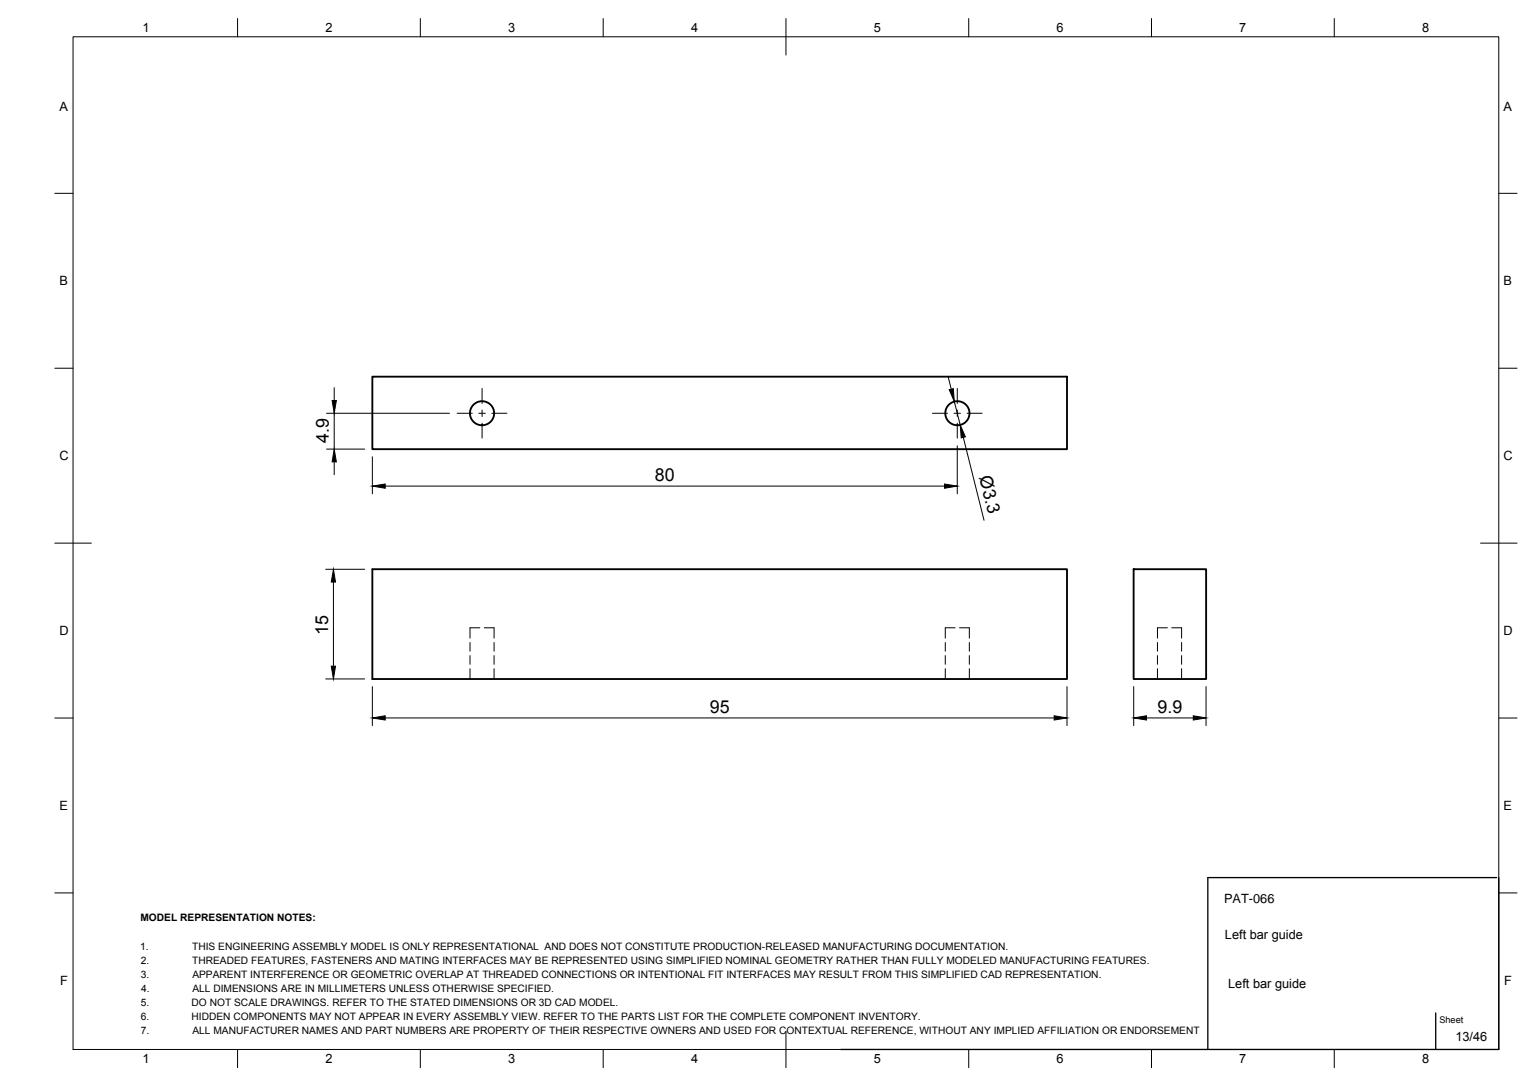
ISO-10303-21;
HEADER;
/* Generated by software containing ST-Developer
 * from STEP Tools, Inc. (www.steptools.com) 
 */

FILE_DESCRIPTION(
/* description */ ('Lever-operated bar clamp (toggle)'),
/* implementation_level */ '2;1');

FILE_NAME(
/* name */ 'Left bar guide.step',
/* time_stamp */ '2026-10-28T03:25:02-07:00',
/* author */ (''),
/* organization */ (''),
/* preprocessor_version */ 'ST-DEVELOPER v20.2',
/* originating_system */ 'Autodesk Translation Framework v15.17.0.0',
/* authorisation */ '');

FILE_SCHEMA (('AUTOMOTIVE_DESIGN { 1 0 10303 214 3 1 1 }'));
ENDSEC;

DATA;
#10=MECHANICAL_DESIGN_GEOMETRIC_PRESENTATION_REPRESENTATION('',(#418),#12413);
#342=SHAPE_REPRESENTATION_RELATIONSHIP('SRR','None',#12581,#380);
#380=ADVANCED_BREP_SHAPE_REPRESENTATION('',(#465),#12378);
#418=STYLED_ITEM('',(#12862),#465);
#465=MANIFOLD_SOLID_BREP('Body1',#6577);
#581=FACE_BOUND('',#1493,.T.);
#582=FACE_BOUND('',#1494,.T.);
#708=PLANE('',#7263);
#709=PLANE('',#7267);
#710=PLANE('',#7268);
#711=PLANE('',#7269);
#712=PLANE('',#7270);
#713=PLANE('',#7271);
#714=PLANE('',#7272);
#715=PLANE('',#7273);
#996=FACE_OUTER_BOUND('',#1483,.T.);
#997=FACE_OUTER_BOUND('',#1484,.T.);
#998=FACE_OUTER_BOUND('',#1485,.T.);
#999=FACE_OUTER_BOUND('',#1486,.T.);
#1000=FACE_OUTER_BOUND('',#1487,.T.);
#1001=FACE_OUTER_BOUND('',#1488,.T.);
#1002=FACE_OUTER_BOUND('',#1489,.T.);
#1003=FACE_OUTER_BOUND('',#1490,.T.);
#1004=FACE_OUTER_BOUND('',#1491,.T.);
#1005=FACE_OUTER_BOUND('',#1492,.T.);
#1483=EDGE_LOOP('',(#4895,#4896,#4897,#4898));
#1484=EDGE_LOOP('',(#4899));
#1485=EDGE_LOOP('',(#4900,#4901,#4902,#4903));
#1486=EDGE_LOOP('',(#4904));
#1487=EDGE_LOOP('',(#4905,#4906,#4907,#4908));
#1488=EDGE_LOOP('',(#4909,#4910,#4911,#4912));
#1489=EDGE_LOOP('',(#4913,#4914,#4915,#4916));
#1490=EDGE_LOOP('',(#4917,#4918,#4919,#4920));
#1491=EDGE_LOOP('',(#4921,#4922,#4923,#4924));
#1492=EDGE_LOOP('',(#4925,#4926,#4927,#4928));
#1493=EDGE_LOOP('',(#4929));
#1494=EDGE_LOOP('',(#4930));
#1986=LINE('',#10563,#2427);
#1987=LINE('',#10570,#2428);
#1988=LINE('',#10576,#2429);
#1989=LINE('',#10578,#2430);
#1990=LINE('',#10580,#2431);
#1991=LINE('',#10581,#2432);
#1992=LINE('',#10584,#2433);
#1993=LINE('',#10586,#2434);
#1994=LINE('',#10587,#2435);
#1995=LINE('',#10590,#2436);
#1996=LINE('',#10592,#2437);
#1997=LINE('',#10593,#2438);
#1998=LINE('',#10595,#2439);
#1999=LINE('',#10596,#2440);
#2427=VECTOR('',#8475,0.165);
#2428=VECTOR('',#8484,0.165);
#2429=VECTOR('',#8491,1.);
#2430=VECTOR('',#8492,1.);
#2431=VECTOR('',#8493,1.);
#2432=VECTOR('',#8494,1.);
#2433=VECTOR('',#8497,1.);
#2434=VECTOR('',#8498,1.);
#2435=VECTOR('',#8499,1.);
#2436=VECTOR('',#8502,1.);
#2437=VECTOR('',#8503,1.);
#2438=VECTOR('',#8504,1.);
#2439=VECTOR('',#8507,1.);
#2440=VECTOR('',#8508,1.);
#2835=CIRCLE('',#7261,0.165);
#2836=CIRCLE('',#7262,0.165);
#2837=CIRCLE('',#7265,0.165);
#2838=CIRCLE('',#7266,0.165);
#3232=VERTEX_POINT('',#10560);
#3233=VERTEX_POINT('',#10562);
#3234=VERTEX_POINT('',#10567);
#3235=VERTEX_POINT('',#10569);
#3236=VERTEX_POINT('',#10574);
#3237=VERTEX_POINT('',#10575);
#3238=VERTEX_POINT('',#10577);
#3239=VERTEX_POINT('',#10579);
#3240=VERTEX_POINT('',#10583);
#3241=VERTEX_POINT('',#10585);
#3242=VERTEX_POINT('',#10589);
#3243=VERTEX_POINT('',#10591);
#3852=EDGE_CURVE('',#3232,#3232,#2835,.T.);
#3853=EDGE_CURVE('',#3232,#3233,#1986,.T.);
#3854=EDGE_CURVE('',#3233,#3233,#2836,.T.);
#3855=EDGE_CURVE('',#3234,#3234,#2837,.T.);
#3856=EDGE_CURVE('',#3234,#3235,#1987,.T.);
#3857=EDGE_CURVE('',#3235,#3235,#2838,.T.);
#3858=EDGE_CURVE('',#3236,#3237,#1988,.T.);
#3859=EDGE_CURVE('',#3237,#3238,#1989,.T.);
#3860=EDGE_CURVE('',#3239,#3238,#1990,.T.);
#3861=EDGE_CURVE('',#3236,#3239,#1991,.T.);
#3862=EDGE_CURVE('',#3240,#3236,#1992,.T.);
#3863=EDGE_CURVE('',#3241,#3239,#1993,.T.);
#3864=EDGE_CURVE('',#3240,#3241,#1994,.T.);
#3865=EDGE_CURVE('',#3242,#3240,#1995,.T.);
#3866=EDGE_CURVE('',#3243,#3241,#1996,.T.);
#3867=EDGE_CURVE('',#3242,#3243,#1997,.T.);
#3868=EDGE_CURVE('',#3237,#3242,#1998,.T.);
#3869=EDGE_CURVE('',#3238,#3243,#1999,.T.);
#4895=ORIENTED_EDGE('',*,*,#3852,.F.);
#4896=ORIENTED_EDGE('',*,*,#3853,.T.);
#4897=ORIENTED_EDGE('',*,*,#3854,.T.);
#4898=ORIENTED_EDGE('',*,*,#3853,.F.);
#4899=ORIENTED_EDGE('',*,*,#3854,.F.);
#4900=ORIENTED_EDGE('',*,*,#3855,.F.);
#4901=ORIENTED_EDGE('',*,*,#3856,.T.);
#4902=ORIENTED_EDGE('',*,*,#3857,.T.);
#4903=ORIENTED_EDGE('',*,*,#3856,.F.);
#4904=ORIENTED_EDGE('',*,*,#3857,.F.);
#4905=ORIENTED_EDGE('',*,*,#3858,.T.);
#4906=ORIENTED_EDGE('',*,*,#3859,.T.);
#4907=ORIENTED_EDGE('',*,*,#3860,.F.);
#4908=ORIENTED_EDGE('',*,*,#3861,.F.);
#4909=ORIENTED_EDGE('',*,*,#3862,.T.);
#4910=ORIENTED_EDGE('',*,*,#3861,.T.);
#4911=ORIENTED_EDGE('',*,*,#3863,.F.);
#4912=ORIENTED_EDGE('',*,*,#3864,.F.);
#4913=ORIENTED_EDGE('',*,*,#3865,.T.);
#4914=ORIENTED_EDGE('',*,*,#3864,.T.);
#4915=ORIENTED_EDGE('',*,*,#3866,.F.);
#4916=ORIENTED_EDGE('',*,*,#3867,.F.);
#4917=ORIENTED_EDGE('',*,*,#3868,.T.);
#4918=ORIENTED_EDGE('',*,*,#3867,.T.);
#4919=ORIENTED_EDGE('',*,*,#3869,.F.);
#4920=ORIENTED_EDGE('',*,*,#3859,.F.);
#4921=ORIENTED_EDGE('',*,*,#3869,.T.);
#4922=ORIENTED_EDGE('',*,*,#3866,.T.);
#4923=ORIENTED_EDGE('',*,*,#3863,.T.);
#4924=ORIENTED_EDGE('',*,*,#3860,.T.);
#4925=ORIENTED_EDGE('',*,*,#3868,.F.);
#4926=ORIENTED_EDGE('',*,*,#3858,.F.);
#4927=ORIENTED_EDGE('',*,*,#3862,.F.);
#4928=ORIENTED_EDGE('',*,*,#3865,.F.);
#4929=ORIENTED_EDGE('',*,*,#3852,.T.);
#4930=ORIENTED_EDGE('',*,*,#3855,.T.);
#6084=CYLINDRICAL_SURFACE('',#7260,0.165);
#6085=CYLINDRICAL_SURFACE('',#7264,0.165);
#6271=ADVANCED_FACE('',(#996),#6084,.F.);
#6272=ADVANCED_FACE('',(#997),#708,.F.);
#6273=ADVANCED_FACE('',(#998),#6085,.F.);
#6274=ADVANCED_FACE('',(#999),#709,.F.);
#6275=ADVANCED_FACE('',(#1000),#710,.T.);
#6276=ADVANCED_FACE('',(#1001),#711,.T.);
#6277=ADVANCED_FACE('',(#1002),#712,.T.);
#6278=ADVANCED_FACE('',(#1003),#713,.T.);
#6279=ADVANCED_FACE('',(#1004),#714,.T.);
#6280=ADVANCED_FACE('',(#1005,#581,#582),#715,.F.);
#6577=CLOSED_SHELL('',(#6271,#6272,#6273,#6274,#6275,#6276,#6277,#6278,
#6279,#6280));
#7259=AXIS2_PLACEMENT_3D('',#10558,#8469,#8470);
#7260=AXIS2_PLACEMENT_3D('',#10559,#8471,#8472);
#7261=AXIS2_PLACEMENT_3D('',#10561,#8473,#8474);
#7262=AXIS2_PLACEMENT_3D('',#10564,#8476,#8477);
#7263=AXIS2_PLACEMENT_3D('',#10565,#8478,#8479);
#7264=AXIS2_PLACEMENT_3D('',#10566,#8480,#8481);
#7265=AXIS2_PLACEMENT_3D('',#10568,#8482,#8483);
#7266=AXIS2_PLACEMENT_3D('',#10571,#8485,#8486);
#7267=AXIS2_PLACEMENT_3D('',#10572,#8487,#8488);
#7268=AXIS2_PLACEMENT_3D('',#10573,#8489,#8490);
#7269=AXIS2_PLACEMENT_3D('',#10582,#8495,#8496);
#7270=AXIS2_PLACEMENT_3D('',#10588,#8500,#8501);
#7271=AXIS2_PLACEMENT_3D('',#10594,#8505,#8506);
#7272=AXIS2_PLACEMENT_3D('',#10597,#8509,#8510);
#7273=AXIS2_PLACEMENT_3D('',#10598,#8511,#8512);
#8469=DIRECTION('axis',(0.,0.,1.));
#8470=DIRECTION('refdir',(1.,0.,0.));
#8471=DIRECTION('center_axis',(0.,0.,1.));
#8472=DIRECTION('ref_axis',(1.,0.,0.));
#8473=DIRECTION('center_axis',(0.,0.,1.));
#8474=DIRECTION('ref_axis',(1.,0.,0.));
#8475=DIRECTION('',(0.,0.,1.));
#8476=DIRECTION('center_axis',(0.,0.,1.));
#8477=DIRECTION('ref_axis',(1.,0.,0.));
#8478=DIRECTION('center_axis',(0.,0.,1.));
#8479=DIRECTION('ref_axis',(1.,0.,0.));
#8480=DIRECTION('center_axis',(0.,0.,1.));
#8481=DIRECTION('ref_axis',(1.,0.,0.));
#8482=DIRECTION('center_axis',(0.,0.,1.));
#8483=DIRECTION('ref_axis',(1.,0.,0.));
#8484=DIRECTION('',(0.,0.,1.));
#8485=DIRECTION('center_axis',(0.,0.,1.));
#8486=DIRECTION('ref_axis',(1.,0.,0.));
#8487=DIRECTION('center_axis',(0.,0.,1.));
#8488=DIRECTION('ref_axis',(1.,0.,0.));
#8489=DIRECTION('center_axis',(0.,1.,0.));
#8490=DIRECTION('ref_axis',(-1.,0.,0.));
#8491=DIRECTION('',(-1.,0.,0.));
#8492=DIRECTION('',(0.,0.,1.));
#8493=DIRECTION('',(-1.,0.,0.));
#8494=DIRECTION('',(0.,0.,1.));
#8495=DIRECTION('center_axis',(1.,0.,0.));
#8496=DIRECTION('ref_axis',(0.,1.,0.));
#8497=DIRECTION('',(0.,1.,0.));
#8498=DIRECTION('',(0.,1.,0.));
#8499=DIRECTION('',(0.,0.,1.));
#8500=DIRECTION('center_axis',(0.,-1.,0.));
#8501=DIRECTION('ref_axis',(1.,0.,0.));
#8502=DIRECTION('',(1.,0.,0.));
#8503=DIRECTION('',(1.,0.,0.));
#8504=DIRECTION('',(0.,0.,1.));
#8505=DIRECTION('center_axis',(-1.,0.,0.));
#8506=DIRECTION('ref_axis',(0.,-1.,0.));
#8507=DIRECTION('',(0.,-1.,0.));
#8508=DIRECTION('',(0.,-1.,0.));
#8509=DIRECTION('center_axis',(0.,0.,1.));
#8510=DIRECTION('ref_axis',(1.,0.,0.));
#8511=DIRECTION('center_axis',(0.,0.,1.));
#8512=DIRECTION('ref_axis',(1.,0.,0.));
#10558=CARTESIAN_POINT('',(0.,0.,0.));
#10559=CARTESIAN_POINT('Origin',(-1.5,-4.5,0.9));
#10560=CARTESIAN_POINT('',(-1.665,-4.5,1.));
#10561=CARTESIAN_POINT('Origin',(-1.5,-4.5,1.));
#10562=CARTESIAN_POINT('',(-1.665,-4.5,1.7));
#10563=CARTESIAN_POINT('',(-1.665,-4.5,0.9));
#10564=CARTESIAN_POINT('Origin',(-1.5,-4.5,1.7));
#10565=CARTESIAN_POINT('Origin',(-1.5,-4.5,1.7));
#10566=CARTESIAN_POINT('Origin',(-1.5,2.,0.9));
#10567=CARTESIAN_POINT('',(-1.665,2.,1.));
#10568=CARTESIAN_POINT('Origin',(-1.5,2.,1.));
#10569=CARTESIAN_POINT('',(-1.665,2.,1.7));
#10570=CARTESIAN_POINT('',(-1.665,2.,0.9));
#10571=CARTESIAN_POINT('Origin',(-1.5,2.,1.7));
#10572=CARTESIAN_POINT('Origin',(-1.5,2.,1.7));
#10573=CARTESIAN_POINT('Origin',(-1.01,3.5,1.));
#10574=CARTESIAN_POINT('',(-1.01,3.5,1.));
#10575=CARTESIAN_POINT('',(-2.,3.5,1.));
#10576=CARTESIAN_POINT('',(-1.01,3.5,1.));
#10577=CARTESIAN_POINT('',(-2.,3.5,2.5));
#10578=CARTESIAN_POINT('',(-2.,3.5,1.));
#10579=CARTESIAN_POINT('',(-1.01,3.5,2.5));
#10580=CARTESIAN_POINT('',(-1.01,3.5,2.5));
#10581=CARTESIAN_POINT('',(-1.01,3.5,1.));
#10582=CARTESIAN_POINT('Origin',(-1.01,-6.,1.));
#10583=CARTESIAN_POINT('',(-1.01,-6.,1.));
#10584=CARTESIAN_POINT('',(-1.01,-6.,1.));
#10585=CARTESIAN_POINT('',(-1.01,-6.,2.5));
#10586=CARTESIAN_POINT('',(-1.01,-6.,2.5));
#10587=CARTESIAN_POINT('',(-1.01,-6.,1.));
#10588=CARTESIAN_POINT('Origin',(-2.,-6.,1.));
#10589=CARTESIAN_POINT('',(-2.,-6.,1.));
#10590=CARTESIAN_POINT('',(-2.,-6.,1.));
#10591=CARTESIAN_POINT('',(-2.,-6.,2.5));
#10592=CARTESIAN_POINT('',(-2.,-6.,2.5));
#10593=CARTESIAN_POINT('',(-2.,-6.,1.));
#10594=CARTESIAN_POINT('Origin',(-2.,3.5,1.));
#10595=CARTESIAN_POINT('',(-2.,3.5,1.));
#10596=CARTESIAN_POINT('',(-2.,3.5,2.5));
#10597=CARTESIAN_POINT('Origin',(-1.505,-1.25,2.5));
#10598=CARTESIAN_POINT('Origin',(-1.505,-1.25,1.));
#12332=UNCERTAINTY_MEASURE_WITH_UNIT(LENGTH_MEASURE(0.001),#12414,
'DISTANCE_ACCURACY_VALUE',
'Maximum model space distance between geometric entities at asserted c
onnectivities');
#12367=UNCERTAINTY_MEASURE_WITH_UNIT(LENGTH_MEASURE(0.001),#12414,
'DISTANCE_ACCURACY_VALUE',
'Maximum model space distance between geometric entities at asserted c
onnectivities');
#12378=(
GEOMETRIC_REPRESENTATION_CONTEXT(3)
GLOBAL_UNCERTAINTY_ASSIGNED_CONTEXT((#12332))
GLOBAL_UNIT_ASSIGNED_CONTEXT((#12414,#12416,#12417))
REPRESENTATION_CONTEXT('','3D')
);
#12413=(
GEOMETRIC_REPRESENTATION_CONTEXT(3)
GLOBAL_UNCERTAINTY_ASSIGNED_CONTEXT((#12367))
GLOBAL_UNIT_ASSIGNED_CONTEXT((#12414,#12416,#12417))
REPRESENTATION_CONTEXT('','3D')
);
#12414=(
LENGTH_UNIT()
NAMED_UNIT(*)
SI_UNIT(.CENTI.,.METRE.)
);
#12416=(
NAMED_UNIT(*)
PLANE_ANGLE_UNIT()
SI_UNIT($,.RADIAN.)
);
#12417=(
NAMED_UNIT(*)
SI_UNIT($,.STERADIAN.)
SOLID_ANGLE_UNIT()
);
#12428=SHAPE_DEFINITION_REPRESENTATION(#12473,#12581);
#12473=PRODUCT_DEFINITION_SHAPE('',$,#12627);
#12581=SHAPE_REPRESENTATION('',(#7259),#12378);
#12616=PRODUCT_DEFINITION_CONTEXT('part definition',#12753,'design');
#12627=PRODUCT_DEFINITION('Left bar guide','Left bar guide',#12672,#12616);
#12672=PRODUCT_DEFINITION_FORMATION('',$,#12765);
#12753=APPLICATION_CONTEXT(
'Core Data for Automotive Mechanical Design Process');
#12754=PRODUCT_CONTEXT('part definition',#12753,'mechanical');
#12765=PRODUCT('Left bar guide','Left bar guide','Left bar guide',(#12754));
#12856=COLOUR_RGB('Sky Blue',0.24,0.69,0.87);
#12857=FILL_AREA_STYLE_COLOUR('',#12856);
#12858=FILL_AREA_STYLE('',(#12857));
#12859=SURFACE_STYLE_FILL_AREA(#12858);
#12860=SURFACE_SIDE_STYLE('',(#12859));
#12861=SURFACE_STYLE_USAGE(.BOTH.,#12860);
#12862=PRESENTATION_STYLE_ASSIGNMENT((#12861));
ENDSEC;
END-ISO-10303-21;
